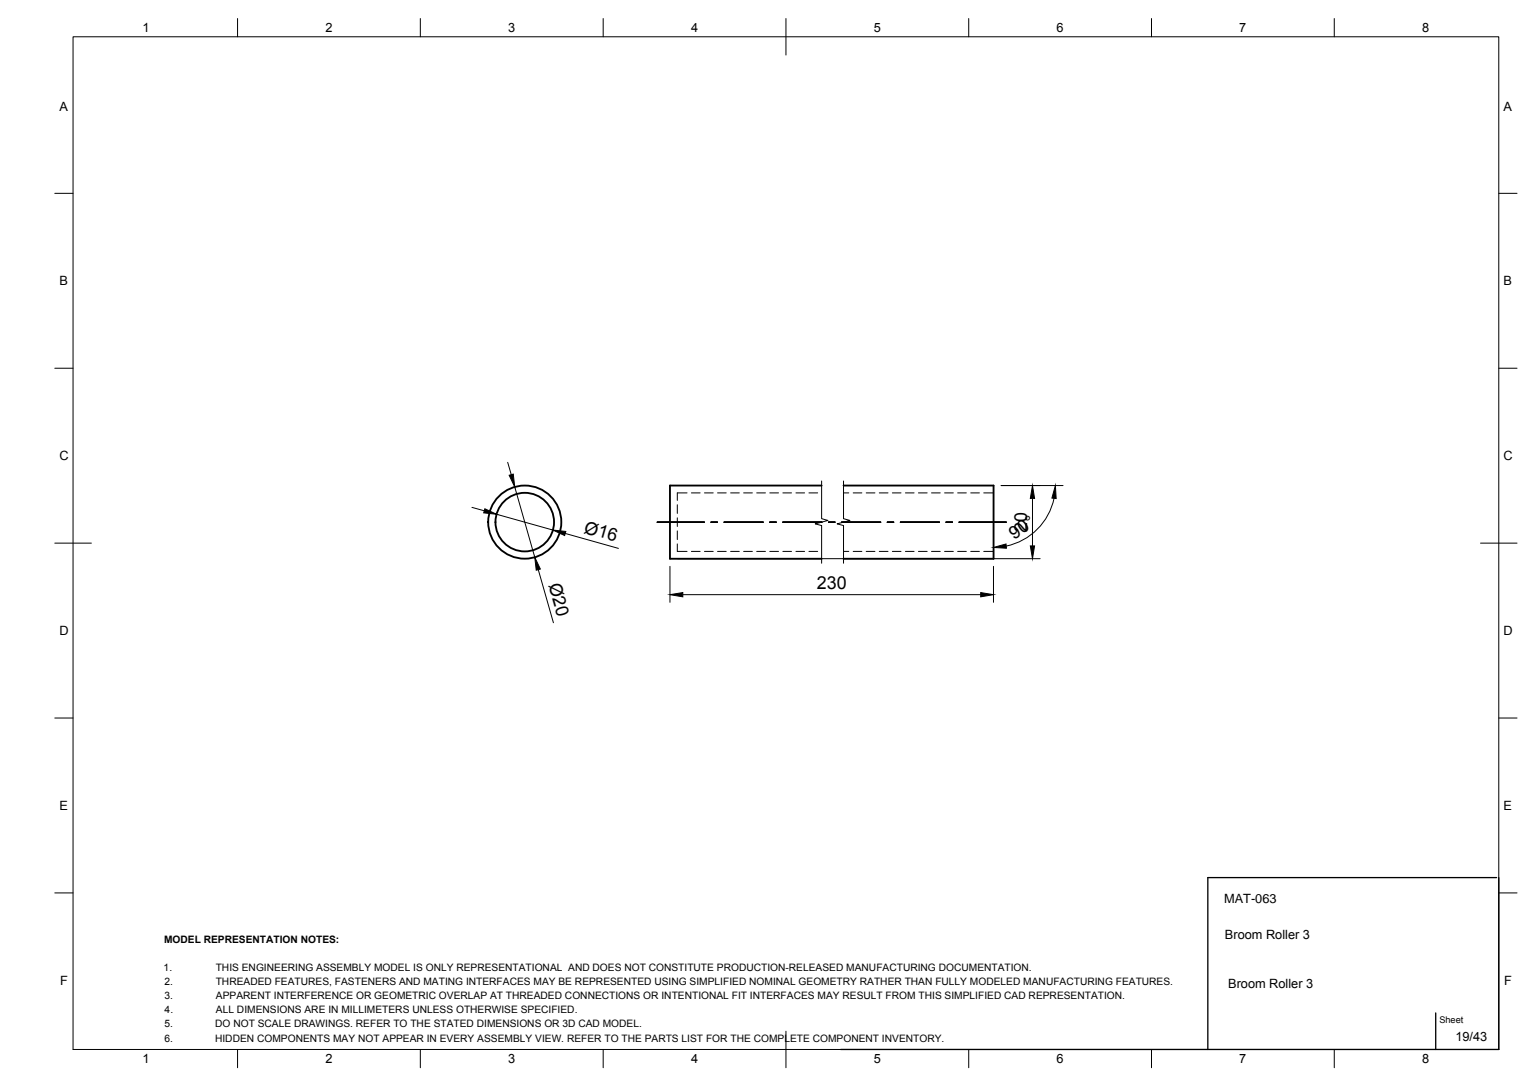
ISO-10303-21;
HEADER;
/* Generated by software containing ST-Developer
 * from STEP Tools, Inc. (www.steptools.com) 
 */

FILE_DESCRIPTION(
/* description */ (''),
/* implementation_level */ '2;1');

FILE_NAME(
/* name */ 'Broom Roller 3.step',
/* time_stamp */ '2026-10-24T09:43:01-07:00',
/* author */ (''),
/* organization */ (''),
/* preprocessor_version */ 'ST-DEVELOPER v20.2',
/* originating_system */ 'Autodesk Translation Framework v15.15.0.0',
/* authorisation */ '');

FILE_SCHEMA (('AUTOMOTIVE_DESIGN { 1 0 10303 214 3 1 1 }'));
ENDSEC;

DATA;
#10=MECHANICAL_DESIGN_GEOMETRIC_PRESENTATION_REPRESENTATION('',(#284),#11112);
#218=SHAPE_REPRESENTATION_RELATIONSHIP('SRR','None',#11242,#251);
#251=ADVANCED_BREP_SHAPE_REPRESENTATION('',(#317),#11087);
#284=STYLED_ITEM('',(#11426),#317);
#317=MANIFOLD_SOLID_BREP('Broom Roller 3',#6021);
#413=FACE_BOUND('',#1296,.T.);
#558=PLANE('',#6864);
#559=PLANE('',#6865);
#560=PLANE('',#6869);
#855=FACE_OUTER_BOUND('',#1293,.T.);
#856=FACE_OUTER_BOUND('',#1294,.T.);
#857=FACE_OUTER_BOUND('',#1295,.T.);
#858=FACE_OUTER_BOUND('',#1297,.T.);
#859=FACE_OUTER_BOUND('',#1298,.T.);
#1293=EDGE_LOOP('',(#4733,#4734,#4735,#4736));
#1294=EDGE_LOOP('',(#4737));
#1295=EDGE_LOOP('',(#4738));
#1296=EDGE_LOOP('',(#4739));
#1297=EDGE_LOOP('',(#4740,#4741,#4742,#4743));
#1298=EDGE_LOOP('',(#4744));
#1690=LINE('',#10161,#2049);
#1691=LINE('',#10170,#2050);
#2049=VECTOR('',#8304,0.00799999959059736);
#2050=VECTOR('',#8317,0.0099999996557502);
#2534=CIRCLE('',#6862,0.00799999959059736);
#2535=CIRCLE('',#6863,0.00799999959059736);
#2536=CIRCLE('',#6866,0.0099999996557502);
#2537=CIRCLE('',#6868,0.0099999996557502);
#2928=VERTEX_POINT('',#10158);
#2929=VERTEX_POINT('',#10160);
#2930=VERTEX_POINT('',#10165);
#2931=VERTEX_POINT('',#10168);
#3570=EDGE_CURVE('',#2928,#2928,#2534,.T.);
#3571=EDGE_CURVE('',#2928,#2929,#1690,.T.);
#3572=EDGE_CURVE('',#2929,#2929,#2535,.F.);
#3573=EDGE_CURVE('',#2930,#2930,#2536,.T.);
#3574=EDGE_CURVE('',#2931,#2931,#2537,.F.);
#3575=EDGE_CURVE('',#2931,#2930,#1691,.T.);
#4733=ORIENTED_EDGE('',*,*,#3570,.F.);
#4734=ORIENTED_EDGE('',*,*,#3571,.T.);
#4735=ORIENTED_EDGE('',*,*,#3572,.F.);
#4736=ORIENTED_EDGE('',*,*,#3571,.F.);
#4737=ORIENTED_EDGE('',*,*,#3572,.T.);
#4738=ORIENTED_EDGE('',*,*,#3573,.F.);
#4739=ORIENTED_EDGE('',*,*,#3570,.T.);
#4740=ORIENTED_EDGE('',*,*,#3574,.T.);
#4741=ORIENTED_EDGE('',*,*,#3575,.T.);
#4742=ORIENTED_EDGE('',*,*,#3573,.T.);
#4743=ORIENTED_EDGE('',*,*,#3575,.F.);
#4744=ORIENTED_EDGE('',*,*,#3574,.F.);
#5571=CYLINDRICAL_SURFACE('',#6861,0.00799999959059736);
#5572=CYLINDRICAL_SURFACE('',#6867,0.0099999996557502);
#5828=ADVANCED_FACE('',(#855),#5571,.F.);
#5829=ADVANCED_FACE('',(#856),#558,.F.);
#5830=ADVANCED_FACE('',(#857,#413),#559,.F.);
#5831=ADVANCED_FACE('',(#858),#5572,.T.);
#5832=ADVANCED_FACE('',(#859),#560,.T.);
#6021=CLOSED_SHELL('',(#5828,#5829,#5830,#5831,#5832));
#6860=AXIS2_PLACEMENT_3D('',#10156,#8298,#8299);
#6861=AXIS2_PLACEMENT_3D('',#10157,#8300,#8301);
#6862=AXIS2_PLACEMENT_3D('',#10159,#8302,#8303);
#6863=AXIS2_PLACEMENT_3D('',#10162,#8305,#8306);
#6864=AXIS2_PLACEMENT_3D('',#10163,#8307,#8308);
#6865=AXIS2_PLACEMENT_3D('',#10164,#8309,#8310);
#6866=AXIS2_PLACEMENT_3D('',#10166,#8311,#8312);
#6867=AXIS2_PLACEMENT_3D('',#10167,#8313,#8314);
#6868=AXIS2_PLACEMENT_3D('',#10169,#8315,#8316);
#6869=AXIS2_PLACEMENT_3D('',#10171,#8318,#8319);
#8298=DIRECTION('axis',(0.,0.,1.));
#8299=DIRECTION('refdir',(1.,0.,0.));
#8300=DIRECTION('center_axis',(0.,-0.388095893070246,0.921618998166817));
#8301=DIRECTION('ref_axis',(0.,-0.921618998166817,-0.388095893070246));
#8302=DIRECTION('center_axis',(0.,-0.388095893070246,0.921618998166817));
#8303=DIRECTION('ref_axis',(0.,-0.921618998166817,-0.388095893070246));
#8304=DIRECTION('',(0.,-0.388095893070246,0.921618998166817));
#8305=DIRECTION('center_axis',(0.,-0.388095893070246,0.921618998166817));
#8306=DIRECTION('ref_axis',(0.,-0.921618998166817,-0.388095893070246));
#8307=DIRECTION('center_axis',(-2.17338651928477E-15,-0.388095852305961,
0.921619015332751));
#8308=DIRECTION('ref_axis',(1.42974172085408E-32,-0.921619015332751,-0.388095852305961));
#8309=DIRECTION('center_axis',(3.34334487188163E-15,-0.388095889853545,
0.921618999521378));
#8310=DIRECTION('ref_axis',(4.30883609996747E-32,-0.921618999521378,-0.388095889853545));
#8311=DIRECTION('center_axis',(0.,-0.388095893070248,0.921618998166817));
#8312=DIRECTION('ref_axis',(0.,-0.921618998166816,-0.388095893070248));
#8313=DIRECTION('center_axis',(0.,-0.388095893070248,0.921618998166817));
#8314=DIRECTION('ref_axis',(0.,-0.921618998166816,-0.388095893070248));
#8315=DIRECTION('center_axis',(0.,-0.388095893070248,0.921618998166817));
#8316=DIRECTION('ref_axis',(0.,-0.921618998166816,-0.388095893070248));
#8317=DIRECTION('',(0.,0.388095893070248,-0.921618998166817));
#8318=DIRECTION('center_axis',(9.77214352076555E-16,-0.388095865559816,
0.921619009751523));
#8319=DIRECTION('ref_axis',(1.19984570551963E-32,-0.921619009751523,-0.388095865559816));
#10156=CARTESIAN_POINT('',(0.,0.,0.));
#10157=CARTESIAN_POINT('Origin',(0.,0.439262055,0.88802763));
#10158=CARTESIAN_POINT('',(-9.79717389180519E-19,0.446635006554106,0.891132397113708));
#10159=CARTESIAN_POINT('Origin',(0.,0.439262054946085,0.888027630128034));
#10160=CARTESIAN_POINT('',(-9.79717389180519E-19,0.358149142877981,1.10126152882899));
#10161=CARTESIAN_POINT('',(-9.79717389180519E-19,0.446635006608021,0.891132396985674));
#10162=CARTESIAN_POINT('Origin',(0.,0.350776191269958,1.09815676184331));
#10163=CARTESIAN_POINT('Origin',(-1.99493199737333E-19,0.3507761915,1.098156762));
#10164=CARTESIAN_POINT('Origin',(-1.56125112837913E-19,0.439262055499997,
0.888027630499999));
#10165=CARTESIAN_POINT('',(-1.22464675698891E-18,0.44847824432875,0.891908589594178));
#10166=CARTESIAN_POINT('Origin',(0.,0.439262054664349,0.888027630797078));
#10167=CARTESIAN_POINT('Origin',(0.,0.439262055,0.88802763));
#10168=CARTESIAN_POINT('',(-1.22464675698891E-18,0.359216189190635,1.10388095853602));
#10169=CARTESIAN_POINT('Origin',(0.,0.349999999526235,1.09999999973892));
#10170=CARTESIAN_POINT('',(-1.22464675698891E-18,0.448478244664401,0.891908588797101));
#10171=CARTESIAN_POINT('Origin',(-1.56125112837913E-19,0.35,1.1));
#11048=UNCERTAINTY_MEASURE_WITH_UNIT(LENGTH_MEASURE(1.E-5),#11113,
'DISTANCE_ACCURACY_VALUE',
'Maximum model space distance between geometric entities at asserted c
onnectivities');
#11073=UNCERTAINTY_MEASURE_WITH_UNIT(LENGTH_MEASURE(1.E-5),#11113,
'DISTANCE_ACCURACY_VALUE',
'Maximum model space distance between geometric entities at asserted c
onnectivities');
#11087=(
GEOMETRIC_REPRESENTATION_CONTEXT(3)
GLOBAL_UNCERTAINTY_ASSIGNED_CONTEXT((#11048))
GLOBAL_UNIT_ASSIGNED_CONTEXT((#11113,#11114,#11115))
REPRESENTATION_CONTEXT('','3D')
);
#11112=(
GEOMETRIC_REPRESENTATION_CONTEXT(3)
GLOBAL_UNCERTAINTY_ASSIGNED_CONTEXT((#11073))
GLOBAL_UNIT_ASSIGNED_CONTEXT((#11113,#11114,#11115))
REPRESENTATION_CONTEXT('','3D')
);
#11113=(
LENGTH_UNIT()
NAMED_UNIT(*)
SI_UNIT($,.METRE.)
);
#11114=(
NAMED_UNIT(*)
PLANE_ANGLE_UNIT()
SI_UNIT($,.RADIAN.)
);
#11115=(
NAMED_UNIT(*)
SI_UNIT($,.STERADIAN.)
SOLID_ANGLE_UNIT()
);
#11129=SHAPE_DEFINITION_REPRESENTATION(#11167,#11242);
#11167=PRODUCT_DEFINITION_SHAPE('',$,#11281);
#11242=SHAPE_REPRESENTATION('',(#6860),#11087);
#11267=PRODUCT_DEFINITION_CONTEXT('part definition',#11383,'design');
#11281=PRODUCT_DEFINITION('Broom Roller 3','Broom Roller 3',#11319,#11267);
#11319=PRODUCT_DEFINITION_FORMATION('',$,#11398);
#11383=APPLICATION_CONTEXT(
'Core Data for Automotive Mechanical Design Process');
#11384=PRODUCT_CONTEXT('part definition',#11383,'mechanical');
#11398=PRODUCT('Broom Roller 3','Broom Roller 3',
'broom_and_roller__ DE     7205',(#11384));
#11426=PRESENTATION_STYLE_ASSIGNMENT((#11430));
#11430=SURFACE_STYLE_USAGE(.BOTH.,#11434);
#11434=SURFACE_SIDE_STYLE('',(#11438));
#11438=SURFACE_STYLE_FILL_AREA(#11442);
#11442=FILL_AREA_STYLE('Opaque(202,209,238)',(#11446));
#11446=FILL_AREA_STYLE_COLOUR('Opaque(202,209,238)',#11450);
#11450=COLOUR_RGB('Opaque(202,209,238)',0.792156862745098,0.819607843137255,
0.933333333333333);
ENDSEC;
END-ISO-10303-21;
